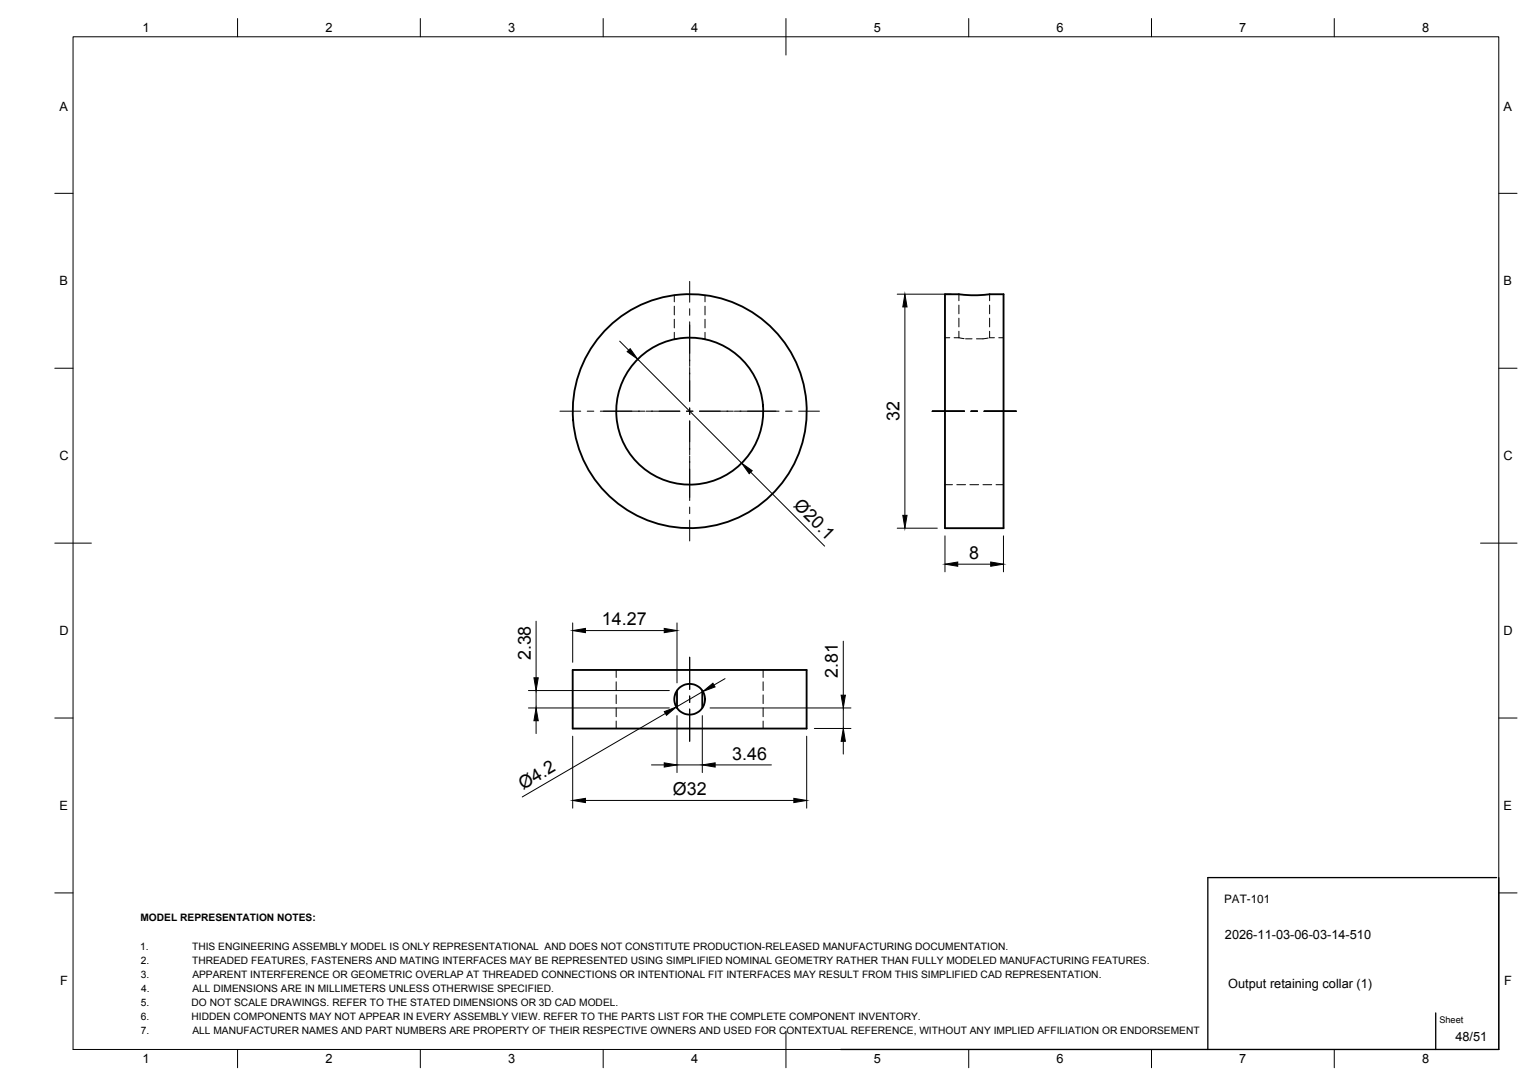
ISO-10303-21;
HEADER;
/* Generated by software containing ST-Developer
 * from STEP Tools, Inc. (www.steptools.com) 
 */

FILE_DESCRIPTION(
/* description */ ('Spur gear reduction stage 2-1 on bearing plates'),
/* implementation_level */ '2;1');

FILE_NAME(
/* name */ 'Output retaining collar (1).step',
/* time_stamp */ '2026-10-28T03:22:07-07:00',
/* author */ (''),
/* organization */ (''),
/* preprocessor_version */ 'ST-DEVELOPER v20.2',
/* originating_system */ 'Autodesk Translation Framework v15.17.0.0',
/* authorisation */ '');

FILE_SCHEMA (('AUTOMOTIVE_DESIGN { 1 0 10303 214 3 1 1 }'));
ENDSEC;

DATA;
#10=MECHANICAL_DESIGN_GEOMETRIC_PRESENTATION_REPRESENTATION('',(#1000),#53909);
#711=B_SPLINE_CURVE_WITH_KNOTS('',3,(#30024,#30025,#30026,#30027,#30028,
#30029,#30030,#30031,#30032,#30033,#30034,#30035,#30036,#30037),
 .UNSPECIFIED.,.F.,.F.,(4,2,2,2,2,2,4),(0.75600573798701,0.793568827564648,
0.872922520054202,0.952276212543757,1.03162990503331,1.11098359752287,1.14854668710051),
 .UNSPECIFIED.);
#712=B_SPLINE_CURVE_WITH_KNOTS('',3,(#30043,#30044,#30045,#30046,#30047,
#30048,#30049,#30050,#30051,#30052,#30053,#30054,#30055,#30056,#30057,#30058,
#30059,#30060),.UNSPECIFIED.,.F.,.F.,(4,2,2,2,2,2,2,2,4),(0.,0.0792028026112442,
0.158405605222488,0.237607602356378,0.316809599490267,0.396011596624156,
0.475213593758045,0.554416396369289,0.633619198980534),.UNSPECIFIED.);
#713=B_SPLINE_CURVE_WITH_KNOTS('',3,(#30061,#30062,#30063,#30064,#30065,
#30066,#30067,#30068,#30069,#30070,#30071,#30072,#30073,#30074,#30075,#30076,
#30077,#30078),.UNSPECIFIED.,.F.,.F.,(4,2,2,2,2,2,2,2,4),(0.633619198980534,
0.712822001591778,0.792024804203022,0.871226801336911,0.9504287984708,1.02963079560469,
1.10883279273858,1.18803559534982,1.26723839796107),.UNSPECIFIED.);
#714=B_SPLINE_CURVE_WITH_KNOTS('',3,(#30081,#30082,#30083,#30084,#30085,
#30086,#30087,#30088,#30089,#30090,#30091,#30092,#30093,#30094),
 .UNSPECIFIED.,.F.,.F.,(4,2,2,2,2,2,4),(0.121154929624506,0.158718019202143,
0.238071711691698,0.317425404181252,0.396779096670807,0.476132789160362,
0.513695878738),.UNSPECIFIED.);
#899=SHAPE_REPRESENTATION_RELATIONSHIP('SRR','None',#54130,#942);
#942=ADVANCED_BREP_SHAPE_REPRESENTATION('',(#1055),#53904);
#1000=STYLED_ITEM('',(#54411),#1055);
#1055=MANIFOLD_SOLID_BREP('Body1',#11327);
#1228=FACE_BOUND('',#2770,.T.);
#1229=FACE_BOUND('',#2772,.T.);
#1230=FACE_BOUND('',#2774,.T.);
#1231=FACE_BOUND('',#2776,.T.);
#1432=PLANE('',#12733);
#1433=PLANE('',#12738);
#1434=PLANE('',#12745);
#1435=PLANE('',#12746);
#1950=FACE_OUTER_BOUND('',#2766,.T.);
#1951=FACE_OUTER_BOUND('',#2767,.T.);
#1952=FACE_OUTER_BOUND('',#2768,.T.);
#1953=FACE_OUTER_BOUND('',#2769,.T.);
#1954=FACE_OUTER_BOUND('',#2771,.T.);
#1955=FACE_OUTER_BOUND('',#2773,.T.);
#1956=FACE_OUTER_BOUND('',#2775,.T.);
#2766=EDGE_LOOP('',(#9288,#9289));
#2767=EDGE_LOOP('',(#9290,#9291,#9292,#9293,#9294,#9295,#9296,#9297,#9298));
#2768=EDGE_LOOP('',(#9299,#9300,#9301));
#2769=EDGE_LOOP('',(#9302,#9303,#9304,#9305));
#2770=EDGE_LOOP('',(#9306,#9307,#9308,#9309));
#2771=EDGE_LOOP('',(#9310,#9311,#9312,#9313));
#2772=EDGE_LOOP('',(#9314,#9315));
#2773=EDGE_LOOP('',(#9316));
#2774=EDGE_LOOP('',(#9317));
#2775=EDGE_LOOP('',(#9318));
#2776=EDGE_LOOP('',(#9319));
#3395=LINE('',#30020,#4036);
#3396=LINE('',#30041,#4037);
#3397=LINE('',#30096,#4038);
#3398=LINE('',#30101,#4039);
#3399=LINE('',#30107,#4040);
#4036=VECTOR('',#15256,1.);
#4037=VECTOR('',#15263,0.21);
#4038=VECTOR('',#15268,1.);
#4039=VECTOR('',#15273,1.005);
#4040=VECTOR('',#15280,1.6);
#4685=CIRCLE('',#12734,0.21);
#4686=CIRCLE('',#12736,0.21);
#4687=CIRCLE('',#12737,0.21);
#4688=CIRCLE('',#12740,1.005);
#4689=CIRCLE('',#12741,1.005);
#4690=CIRCLE('',#12743,1.6);
#4691=CIRCLE('',#12744,1.6);
#5441=VERTEX_POINT('',#30018);
#5442=VERTEX_POINT('',#30019);
#5443=VERTEX_POINT('',#30023);
#5444=VERTEX_POINT('',#30038);
#5445=VERTEX_POINT('',#30040);
#5446=VERTEX_POINT('',#30042);
#5447=VERTEX_POINT('',#30079);
#5448=VERTEX_POINT('',#30098);
#5449=VERTEX_POINT('',#30100);
#5450=VERTEX_POINT('',#30104);
#5451=VERTEX_POINT('',#30106);
#6786=EDGE_CURVE('',#5441,#5442,#3395,.T.);
#6787=EDGE_CURVE('',#5441,#5442,#4685,.T.);
#6788=EDGE_CURVE('',#5443,#5441,#711,.T.);
#6789=EDGE_CURVE('',#5444,#5443,#4686,.T.);
#6790=EDGE_CURVE('',#5444,#5445,#3396,.T.);
#6791=EDGE_CURVE('',#5446,#5445,#712,.T.);
#6792=EDGE_CURVE('',#5445,#5446,#713,.T.);
#6793=EDGE_CURVE('',#5447,#5444,#4687,.T.);
#6794=EDGE_CURVE('',#5442,#5447,#714,.T.);
#6795=EDGE_CURVE('',#5447,#5443,#3397,.T.);
#6796=EDGE_CURVE('',#5448,#5448,#4688,.T.);
#6797=EDGE_CURVE('',#5448,#5449,#3398,.T.);
#6798=EDGE_CURVE('',#5449,#5449,#4689,.T.);
#6799=EDGE_CURVE('',#5450,#5450,#4690,.T.);
#6800=EDGE_CURVE('',#5450,#5451,#3399,.T.);
#6801=EDGE_CURVE('',#5451,#5451,#4691,.T.);
#9288=ORIENTED_EDGE('',*,*,#6786,.F.);
#9289=ORIENTED_EDGE('',*,*,#6787,.T.);
#9290=ORIENTED_EDGE('',*,*,#6788,.F.);
#9291=ORIENTED_EDGE('',*,*,#6789,.F.);
#9292=ORIENTED_EDGE('',*,*,#6790,.T.);
#9293=ORIENTED_EDGE('',*,*,#6791,.F.);
#9294=ORIENTED_EDGE('',*,*,#6792,.F.);
#9295=ORIENTED_EDGE('',*,*,#6790,.F.);
#9296=ORIENTED_EDGE('',*,*,#6793,.F.);
#9297=ORIENTED_EDGE('',*,*,#6794,.F.);
#9298=ORIENTED_EDGE('',*,*,#6787,.F.);
#9299=ORIENTED_EDGE('',*,*,#6795,.F.);
#9300=ORIENTED_EDGE('',*,*,#6793,.T.);
#9301=ORIENTED_EDGE('',*,*,#6789,.T.);
#9302=ORIENTED_EDGE('',*,*,#6796,.F.);
#9303=ORIENTED_EDGE('',*,*,#6797,.T.);
#9304=ORIENTED_EDGE('',*,*,#6798,.T.);
#9305=ORIENTED_EDGE('',*,*,#6797,.F.);
#9306=ORIENTED_EDGE('',*,*,#6794,.T.);
#9307=ORIENTED_EDGE('',*,*,#6795,.T.);
#9308=ORIENTED_EDGE('',*,*,#6788,.T.);
#9309=ORIENTED_EDGE('',*,*,#6786,.T.);
#9310=ORIENTED_EDGE('',*,*,#6799,.F.);
#9311=ORIENTED_EDGE('',*,*,#6800,.T.);
#9312=ORIENTED_EDGE('',*,*,#6801,.T.);
#9313=ORIENTED_EDGE('',*,*,#6800,.F.);
#9314=ORIENTED_EDGE('',*,*,#6791,.T.);
#9315=ORIENTED_EDGE('',*,*,#6792,.T.);
#9316=ORIENTED_EDGE('',*,*,#6799,.T.);
#9317=ORIENTED_EDGE('',*,*,#6796,.T.);
#9318=ORIENTED_EDGE('',*,*,#6801,.F.);
#9319=ORIENTED_EDGE('',*,*,#6798,.F.);
#10575=CYLINDRICAL_SURFACE('',#12735,0.21);
#10576=CYLINDRICAL_SURFACE('',#12739,1.005);
#10577=CYLINDRICAL_SURFACE('',#12742,1.6);
#11070=ADVANCED_FACE('',(#1950),#1432,.T.);
#11071=ADVANCED_FACE('',(#1951),#10575,.F.);
#11072=ADVANCED_FACE('',(#1952),#1433,.T.);
#11073=ADVANCED_FACE('',(#1953,#1228),#10576,.F.);
#11074=ADVANCED_FACE('',(#1954,#1229),#10577,.T.);
#11075=ADVANCED_FACE('',(#1955,#1230),#1434,.T.);
#11076=ADVANCED_FACE('',(#1956,#1231),#1435,.F.);
#11327=CLOSED_SHELL('',(#11070,#11071,#11072,#11073,#11074,#11075,#11076));
#12732=AXIS2_PLACEMENT_3D('',#30016,#15252,#15253);
#12733=AXIS2_PLACEMENT_3D('',#30017,#15254,#15255);
#12734=AXIS2_PLACEMENT_3D('',#30021,#15257,#15258);
#12735=AXIS2_PLACEMENT_3D('',#30022,#15259,#15260);
#12736=AXIS2_PLACEMENT_3D('',#30039,#15261,#15262);
#12737=AXIS2_PLACEMENT_3D('',#30080,#15264,#15265);
#12738=AXIS2_PLACEMENT_3D('',#30095,#15266,#15267);
#12739=AXIS2_PLACEMENT_3D('',#30097,#15269,#15270);
#12740=AXIS2_PLACEMENT_3D('',#30099,#15271,#15272);
#12741=AXIS2_PLACEMENT_3D('',#30102,#15274,#15275);
#12742=AXIS2_PLACEMENT_3D('',#30103,#15276,#15277);
#12743=AXIS2_PLACEMENT_3D('',#30105,#15278,#15279);
#12744=AXIS2_PLACEMENT_3D('',#30108,#15281,#15282);
#12745=AXIS2_PLACEMENT_3D('',#30109,#15283,#15284);
#12746=AXIS2_PLACEMENT_3D('',#30110,#15285,#15286);
#15252=DIRECTION('axis',(0.,0.,1.));
#15253=DIRECTION('refdir',(1.,0.,0.));
#15254=DIRECTION('center_axis',(0.,0.,1.));
#15255=DIRECTION('ref_axis',(1.,0.,0.));
#15256=DIRECTION('',(0.,1.,0.));
#15257=DIRECTION('center_axis',(0.,0.,1.));
#15258=DIRECTION('ref_axis',(1.,0.,0.));
#15259=DIRECTION('center_axis',(0.,0.,1.));
#15260=DIRECTION('ref_axis',(1.,0.,0.));
#15261=DIRECTION('center_axis',(0.,0.,1.));
#15262=DIRECTION('ref_axis',(1.,0.,0.));
#15263=DIRECTION('',(0.,0.,1.));
#15264=DIRECTION('center_axis',(0.,0.,1.));
#15265=DIRECTION('ref_axis',(1.,0.,0.));
#15266=DIRECTION('center_axis',(0.,0.,1.));
#15267=DIRECTION('ref_axis',(1.,0.,0.));
#15268=DIRECTION('',(0.,-1.,0.));
#15269=DIRECTION('center_axis',(0.,1.,0.));
#15270=DIRECTION('ref_axis',(1.,0.,0.));
#15271=DIRECTION('center_axis',(0.,-1.,0.));
#15272=DIRECTION('ref_axis',(1.,0.,0.));
#15273=DIRECTION('',(0.,-1.,0.));
#15274=DIRECTION('center_axis',(0.,-1.,0.));
#15275=DIRECTION('ref_axis',(1.,0.,0.));
#15276=DIRECTION('center_axis',(0.,1.,0.));
#15277=DIRECTION('ref_axis',(1.,0.,0.));
#15278=DIRECTION('center_axis',(0.,1.,0.));
#15279=DIRECTION('ref_axis',(1.,0.,0.));
#15280=DIRECTION('',(0.,-1.,0.));
#15281=DIRECTION('center_axis',(0.,1.,0.));
#15282=DIRECTION('ref_axis',(1.,0.,0.));
#15283=DIRECTION('center_axis',(0.,1.,0.));
#15284=DIRECTION('ref_axis',(1.,0.,0.));
#15285=DIRECTION('center_axis',(0.,1.,0.));
#15286=DIRECTION('ref_axis',(1.,0.,0.));
#30016=CARTESIAN_POINT('',(0.,0.,0.));
#30017=CARTESIAN_POINT('Origin',(0.,5.1,0.99));
#30018=CARTESIAN_POINT('',(0.172988438920062,4.98094119100209,0.99));
#30019=CARTESIAN_POINT('',(0.172988438920062,5.21905880899791,0.99));
#30020=CARTESIAN_POINT('',(0.172988438920062,4.7,0.99));
#30021=CARTESIAN_POINT('Origin',(0.,5.1,0.99));
#30022=CARTESIAN_POINT('Origin',(0.,5.1,0.99));
#30023=CARTESIAN_POINT('',(-0.172988438920062,4.98094119100209,0.99));
#30024=CARTESIAN_POINT('Ctrl Pts',(-0.172988438920062,4.98094119100209,
0.99));
#30025=CARTESIAN_POINT('Ctrl Pts',(-0.165594865311318,4.97019857760471,
0.991291921976381));
#30026=CARTESIAN_POINT('Ctrl Pts',(-0.157297138725609,4.96031229062726,
0.992653949439047));
#30027=CARTESIAN_POINT('Ctrl Pts',(-0.129892073845076,4.93290722574673,
0.996748084390898));
#30028=CARTESIAN_POINT('Ctrl Pts',(-0.106330167759284,4.91675794366705,
0.999695893276376));
#30029=CARTESIAN_POINT('Ctrl Pts',(-0.05461290463241,4.89530220603509,1.00385029472357));
#30030=CARTESIAN_POINT('Ctrl Pts',(-0.0264512308298516,4.89,1.005));
#30031=CARTESIAN_POINT('Ctrl Pts',(0.0264512308298516,4.89,1.005));
#30032=CARTESIAN_POINT('Ctrl Pts',(0.0546129046324099,4.89530220603509,
1.00385029472357));
#30033=CARTESIAN_POINT('Ctrl Pts',(0.106330167759284,4.91675794366705,0.999695893276376));
#30034=CARTESIAN_POINT('Ctrl Pts',(0.129892073845076,4.93290722574673,0.996748084390898));
#30035=CARTESIAN_POINT('Ctrl Pts',(0.157297138725609,4.96031229062726,0.992653949439047));
#30036=CARTESIAN_POINT('Ctrl Pts',(0.165594865311318,4.97019857760471,0.991291921976381));
#30037=CARTESIAN_POINT('Ctrl Pts',(0.172988438920062,4.98094119100209,0.99));
#30038=CARTESIAN_POINT('',(-0.21,5.1,0.99));
#30039=CARTESIAN_POINT('Origin',(0.,5.1,0.99));
#30040=CARTESIAN_POINT('',(-0.21,5.1,1.58615888233178));
#30041=CARTESIAN_POINT('',(-0.21,5.1,0.99));
#30042=CARTESIAN_POINT('',(0.21,5.1,1.58615888233178));
#30043=CARTESIAN_POINT('Ctrl Pts',(0.21,5.1,1.58615888233178));
#30044=CARTESIAN_POINT('Ctrl Pts',(0.21,5.07359906579625,1.58615888233178));
#30045=CARTESIAN_POINT('Ctrl Pts',(0.20471752266132,5.04545944463489,1.58688606295397));
#30046=CARTESIAN_POINT('Ctrl Pts',(0.183276841782292,4.9937289476995,1.58950502964782));
#30047=CARTESIAN_POINT('Ctrl Pts',(0.167120287247804,4.97013543914945,1.59135816887013));
#30048=CARTESIAN_POINT('Ctrl Pts',(0.129864750292352,4.932879902194,1.59483075953278));
#30049=CARTESIAN_POINT('Ctrl Pts',(0.106271159541076,4.91672319916876,1.59667690933009));
#30050=CARTESIAN_POINT('Ctrl Pts',(0.0545403836274689,4.8952824096556,1.59927985626981));
#30051=CARTESIAN_POINT('Ctrl Pts',(0.0264006657112964,4.89,1.6));
#30052=CARTESIAN_POINT('Ctrl Pts',(-0.0264006657112964,4.89,1.6));
#30053=CARTESIAN_POINT('Ctrl Pts',(-0.0545403836274688,4.8952824096556,
1.59927985626981));
#30054=CARTESIAN_POINT('Ctrl Pts',(-0.106271159541076,4.91672319916876,
1.59667690933009));
#30055=CARTESIAN_POINT('Ctrl Pts',(-0.129864750292352,4.932879902194,1.59483075953278));
#30056=CARTESIAN_POINT('Ctrl Pts',(-0.167120287247804,4.97013543914945,
1.59135816887013));
#30057=CARTESIAN_POINT('Ctrl Pts',(-0.183276841782292,4.9937289476995,1.58950502964782));
#30058=CARTESIAN_POINT('Ctrl Pts',(-0.20471752266132,5.04545944463489,1.58688606295397));
#30059=CARTESIAN_POINT('Ctrl Pts',(-0.21,5.07359906579625,1.58615888233178));
#30060=CARTESIAN_POINT('Ctrl Pts',(-0.21,5.1,1.58615888233178));
#30061=CARTESIAN_POINT('Ctrl Pts',(-0.21,5.1,1.58615888233178));
#30062=CARTESIAN_POINT('Ctrl Pts',(-0.21,5.12640093420375,1.58615888233178));
#30063=CARTESIAN_POINT('Ctrl Pts',(-0.20471752266132,5.15454055536511,1.58688606295397));
#30064=CARTESIAN_POINT('Ctrl Pts',(-0.183276841782292,5.2062710523005,1.58950502964782));
#30065=CARTESIAN_POINT('Ctrl Pts',(-0.167120287247804,5.22986456085055,
1.59135816887013));
#30066=CARTESIAN_POINT('Ctrl Pts',(-0.129864750292352,5.267120097806,1.59483075953278));
#30067=CARTESIAN_POINT('Ctrl Pts',(-0.106271159541076,5.28327680083123,
1.59667690933009));
#30068=CARTESIAN_POINT('Ctrl Pts',(-0.0545403836274689,5.3047175903444,
1.59927985626981));
#30069=CARTESIAN_POINT('Ctrl Pts',(-0.0264006657112965,5.31,1.6));
#30070=CARTESIAN_POINT('Ctrl Pts',(0.0264006657112964,5.31,1.6));
#30071=CARTESIAN_POINT('Ctrl Pts',(0.0545403836274689,5.3047175903444,1.59927985626981));
#30072=CARTESIAN_POINT('Ctrl Pts',(0.106271159541076,5.28327680083123,1.59667690933009));
#30073=CARTESIAN_POINT('Ctrl Pts',(0.129864750292352,5.267120097806,1.59483075953278));
#30074=CARTESIAN_POINT('Ctrl Pts',(0.167120287247804,5.22986456085055,1.59135816887013));
#30075=CARTESIAN_POINT('Ctrl Pts',(0.183276841782292,5.2062710523005,1.58950502964782));
#30076=CARTESIAN_POINT('Ctrl Pts',(0.20471752266132,5.15454055536511,1.58688606295397));
#30077=CARTESIAN_POINT('Ctrl Pts',(0.21,5.12640093420375,1.58615888233178));
#30078=CARTESIAN_POINT('Ctrl Pts',(0.21,5.1,1.58615888233178));
#30079=CARTESIAN_POINT('',(-0.172988438920062,5.21905880899791,0.99));
#30080=CARTESIAN_POINT('Origin',(0.,5.1,0.99));
#30081=CARTESIAN_POINT('Ctrl Pts',(0.172988438920062,5.21905880899791,0.99));
#30082=CARTESIAN_POINT('Ctrl Pts',(0.165594865311319,5.22980142239529,0.991291921976381));
#30083=CARTESIAN_POINT('Ctrl Pts',(0.157297138725609,5.23968770937274,0.992653949439047));
#30084=CARTESIAN_POINT('Ctrl Pts',(0.129892073845076,5.26709277425327,0.996748084390898));
#30085=CARTESIAN_POINT('Ctrl Pts',(0.106330167759284,5.28324205633295,0.999695893276376));
#30086=CARTESIAN_POINT('Ctrl Pts',(0.05461290463241,5.30469779396491,1.00385029472357));
#30087=CARTESIAN_POINT('Ctrl Pts',(0.0264512308298516,5.31,1.005));
#30088=CARTESIAN_POINT('Ctrl Pts',(-0.0264512308298516,5.31,1.005));
#30089=CARTESIAN_POINT('Ctrl Pts',(-0.0546129046324098,5.30469779396491,
1.00385029472357));
#30090=CARTESIAN_POINT('Ctrl Pts',(-0.106330167759284,5.28324205633295,
0.999695893276376));
#30091=CARTESIAN_POINT('Ctrl Pts',(-0.129892073845076,5.26709277425327,
0.996748084390898));
#30092=CARTESIAN_POINT('Ctrl Pts',(-0.157297138725609,5.23968770937274,
0.992653949439047));
#30093=CARTESIAN_POINT('Ctrl Pts',(-0.165594865311318,5.22980142239529,
0.991291921976381));
#30094=CARTESIAN_POINT('Ctrl Pts',(-0.172988438920062,5.21905880899791,
0.99));
#30095=CARTESIAN_POINT('Origin',(0.,5.1,0.99));
#30096=CARTESIAN_POINT('',(-0.172988438920062,4.7,0.99));
#30097=CARTESIAN_POINT('Origin',(0.,4.7,0.));
#30098=CARTESIAN_POINT('',(-1.005,5.5,1.23077003314309E-16));
#30099=CARTESIAN_POINT('Origin',(0.,5.5,0.));
#30100=CARTESIAN_POINT('',(-1.005,4.7,1.23077003314309E-16));
#30101=CARTESIAN_POINT('',(-1.005,4.7,1.23077003314309E-16));
#30102=CARTESIAN_POINT('Origin',(0.,4.7,0.));
#30103=CARTESIAN_POINT('Origin',(0.,4.7,0.));
#30104=CARTESIAN_POINT('',(-1.6,5.5,1.95943487863577E-16));
#30105=CARTESIAN_POINT('Origin',(0.,5.5,0.));
#30106=CARTESIAN_POINT('',(-1.6,4.7,1.95943487863577E-16));
#30107=CARTESIAN_POINT('',(-1.6,4.7,1.95943487863577E-16));
#30108=CARTESIAN_POINT('Origin',(0.,4.7,0.));
#30109=CARTESIAN_POINT('Origin',(0.,5.5,0.));
#30110=CARTESIAN_POINT('Origin',(0.,4.7,0.));
#53854=UNCERTAINTY_MEASURE_WITH_UNIT(LENGTH_MEASURE(0.001),#53910,
'DISTANCE_ACCURACY_VALUE',
'Maximum model space distance between geometric entities at asserted c
onnectivities');
#53859=UNCERTAINTY_MEASURE_WITH_UNIT(LENGTH_MEASURE(0.001),#53910,
'DISTANCE_ACCURACY_VALUE',
'Maximum model space distance between geometric entities at asserted c
onnectivities');
#53904=(
GEOMETRIC_REPRESENTATION_CONTEXT(3)
GLOBAL_UNCERTAINTY_ASSIGNED_CONTEXT((#53854))
GLOBAL_UNIT_ASSIGNED_CONTEXT((#53910,#53912,#53913))
REPRESENTATION_CONTEXT('','3D')
);
#53909=(
GEOMETRIC_REPRESENTATION_CONTEXT(3)
GLOBAL_UNCERTAINTY_ASSIGNED_CONTEXT((#53859))
GLOBAL_UNIT_ASSIGNED_CONTEXT((#53910,#53912,#53913))
REPRESENTATION_CONTEXT('','3D')
);
#53910=(
LENGTH_UNIT()
NAMED_UNIT(*)
SI_UNIT(.CENTI.,.METRE.)
);
#53912=(
NAMED_UNIT(*)
PLANE_ANGLE_UNIT()
SI_UNIT($,.RADIAN.)
);
#53913=(
NAMED_UNIT(*)
SI_UNIT($,.STERADIAN.)
SOLID_ANGLE_UNIT()
);
#53958=SHAPE_DEFINITION_REPRESENTATION(#54056,#54130);
#54056=PRODUCT_DEFINITION_SHAPE('',$,#54180);
#54130=SHAPE_REPRESENTATION('',(#12732),#53904);
#54135=PRODUCT_DEFINITION_CONTEXT('part definition',#54284,'design');
#54180=PRODUCT_DEFINITION('Output retaining collar (1)',
'Output retaining collar (1)',#54229,#54135);
#54229=PRODUCT_DEFINITION_FORMATION('',$,#54330);
#54284=APPLICATION_CONTEXT(
'Core Data for Automotive Mechanical Design Process');
#54285=PRODUCT_CONTEXT('part definition',#54284,'mechanical');
#54330=PRODUCT('Output retaining collar (1)',
'Output retaining collar (1)','Output retaining collar (1)',(#54285));
#54405=COLOUR_RGB('Off White',0.89,0.88,0.83);
#54406=FILL_AREA_STYLE_COLOUR('',#54405);
#54407=FILL_AREA_STYLE('',(#54406));
#54408=SURFACE_STYLE_FILL_AREA(#54407);
#54409=SURFACE_SIDE_STYLE('',(#54408));
#54410=SURFACE_STYLE_USAGE(.BOTH.,#54409);
#54411=PRESENTATION_STYLE_ASSIGNMENT((#54410));
ENDSEC;
END-ISO-10303-21;
